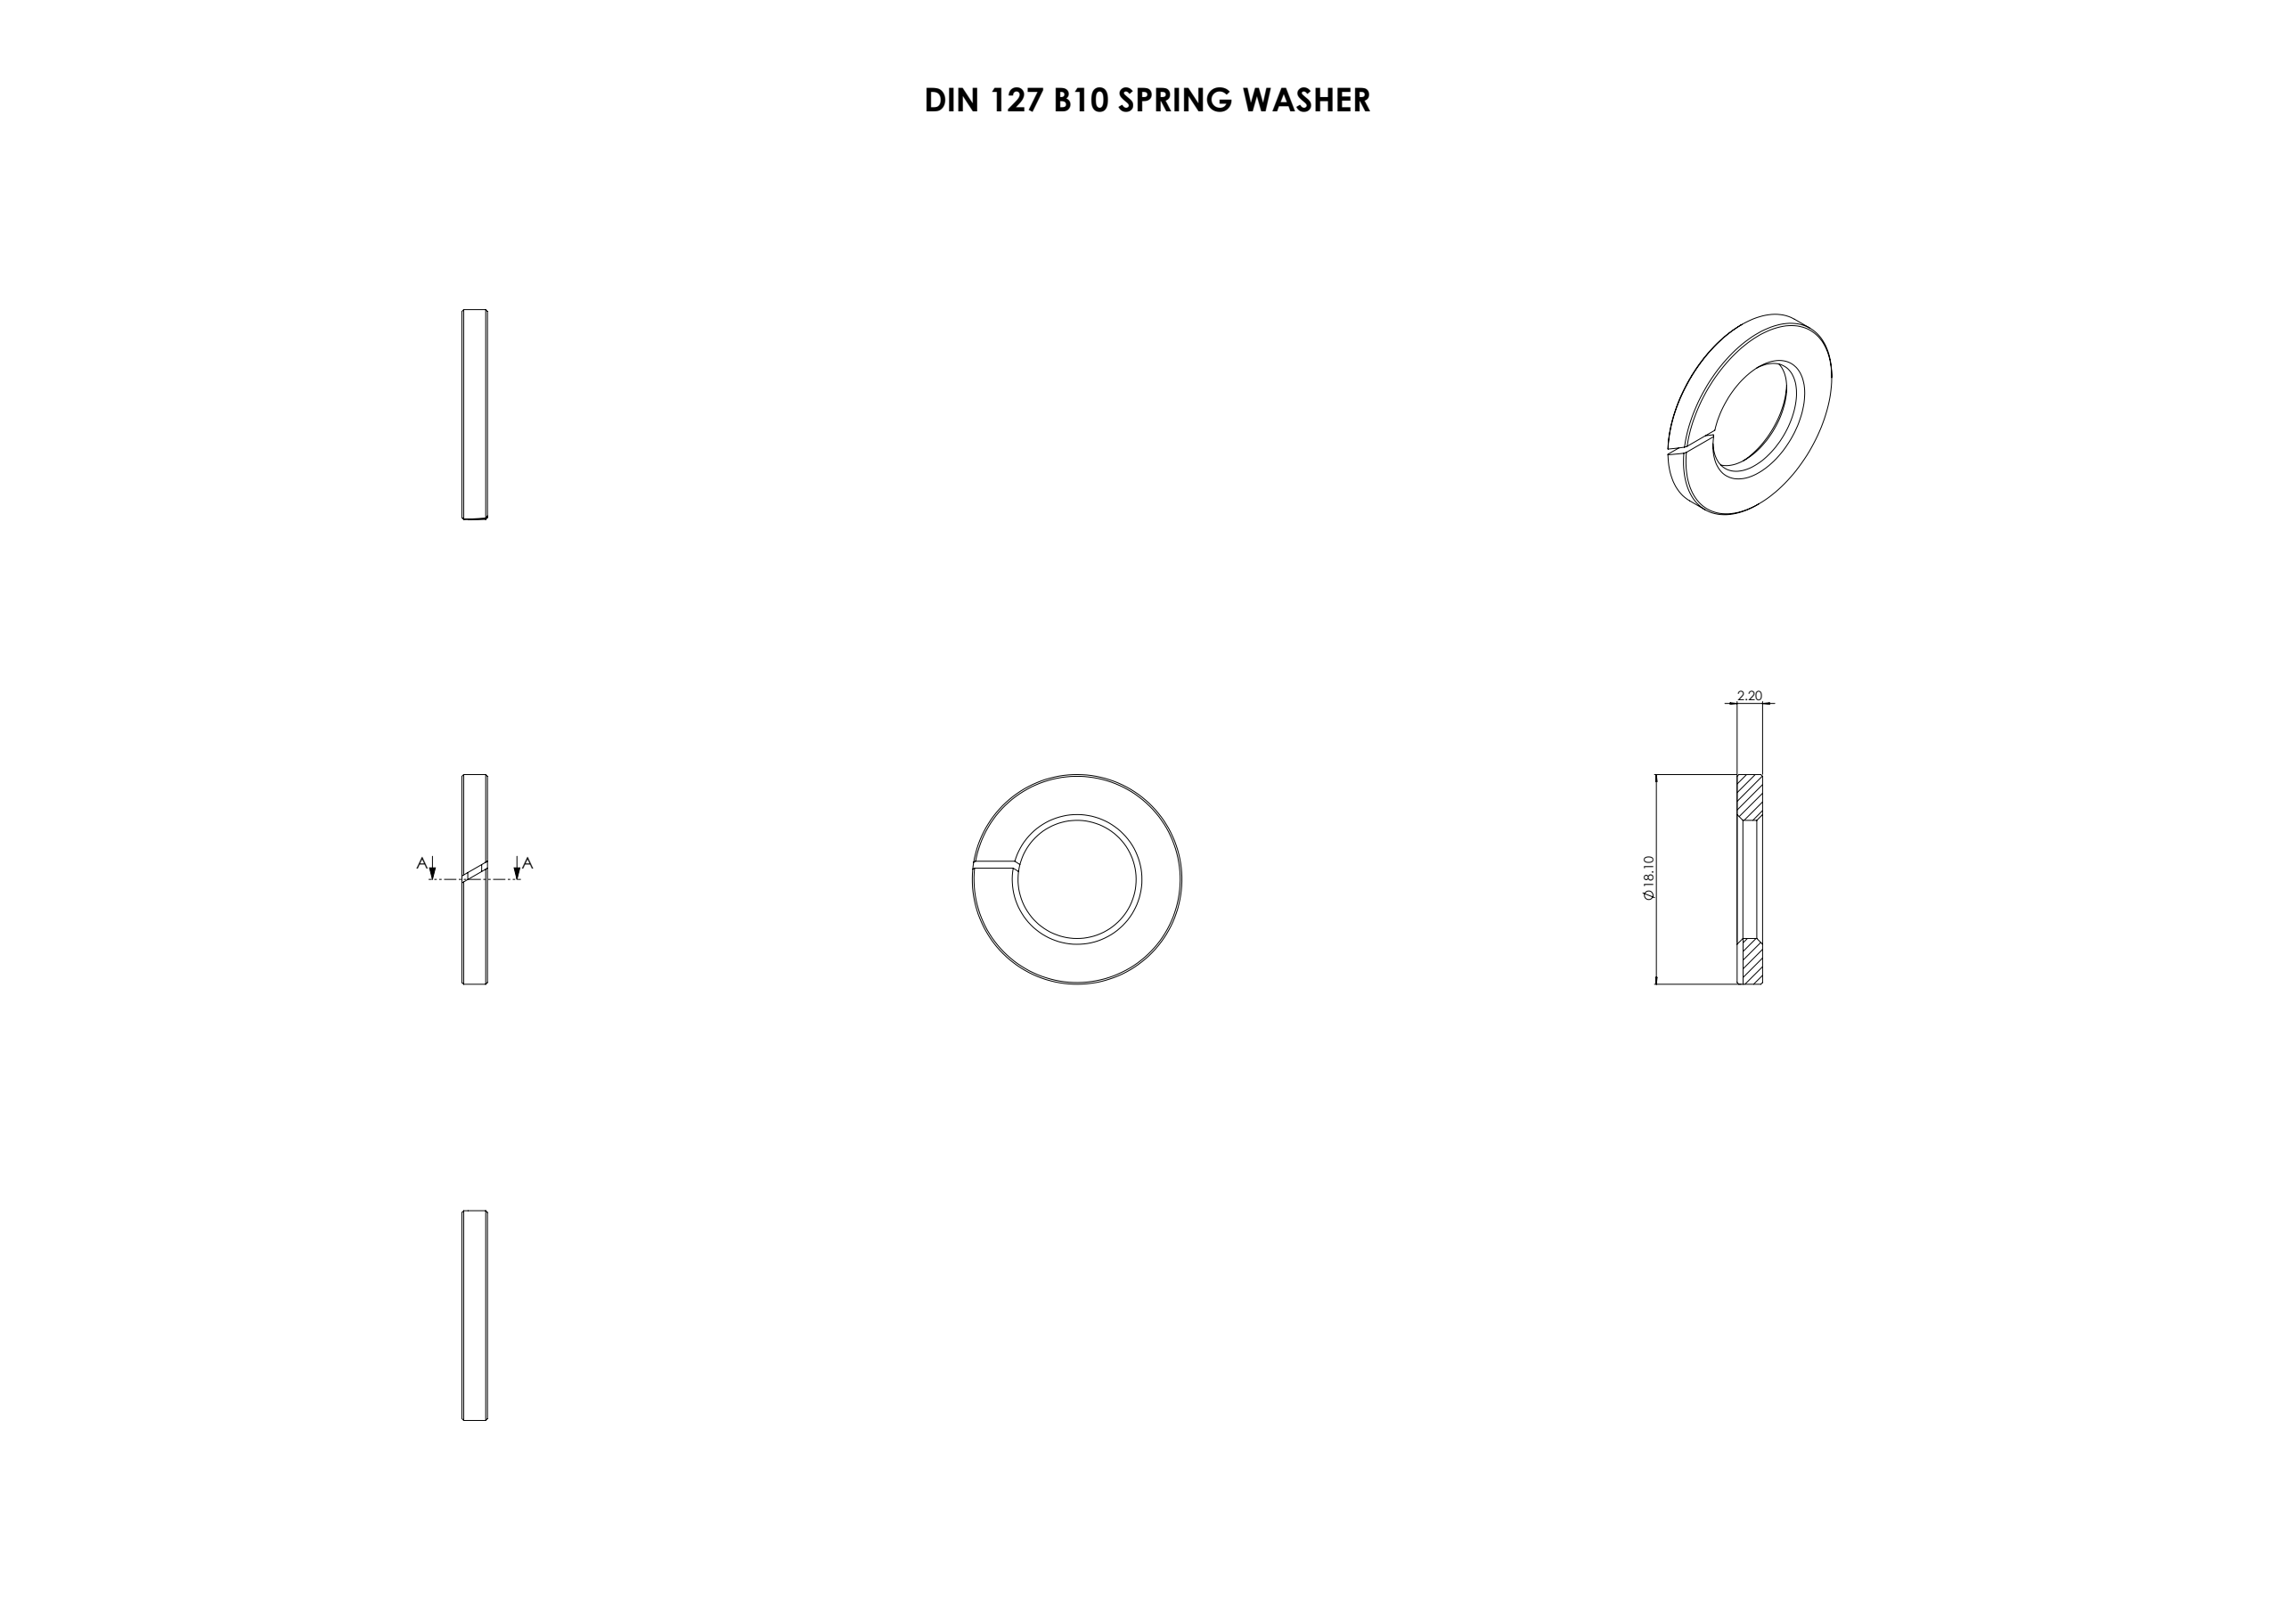
ISO-10303-21;
HEADER;
/* Generated by software containing ST-Developer
 * from STEP Tools, Inc. (www.steptools.com) 
 */

FILE_DESCRIPTION(
/* description */ (''),
/* implementation_level */ '2;1');

FILE_NAME(
/* name */ '08_DIN_127_B10_Spring_Washer.step',
/* time_stamp */ '2026-10-11T08:27:52-07:00',
/* author */ (''),
/* organization */ (''),
/* preprocessor_version */ 'ST-DEVELOPER v20.2',
/* originating_system */ 'Autodesk Translation Framework v15.15.0.0',
/* authorisation */ '');

FILE_SCHEMA (('AUTOMOTIVE_DESIGN { 1 0 10303 214 3 1 1 }'));
ENDSEC;

DATA;
#10=MECHANICAL_DESIGN_GEOMETRIC_PRESENTATION_REPRESENTATION('',(#926),#94301);
#898=SHAPE_REPRESENTATION_RELATIONSHIP('SRR','None',#94378,#912);
#912=ADVANCED_BREP_SHAPE_REPRESENTATION('',(#940),#94294);
#926=STYLED_ITEM('',(#94588),#940);
#940=MANIFOLD_SOLID_BREP('Body1',#51025);
#1194=CYLINDRICAL_SURFACE('',#54830,5.1);
#1195=CYLINDRICAL_SURFACE('',#54834,9.05);
#1196=CYLINDRICAL_SURFACE('',#54845,9.05);
#1197=CYLINDRICAL_SURFACE('',#54853,5.1);
#2152=ELLIPSE('',#54832,10.2,5.1);
#2153=ELLIPSE('',#54836,18.1,9.05);
#2154=ELLIPSE('',#54839,18.1,9.05);
#2155=ELLIPSE('',#54841,10.2,5.1);
#6291=LINE('',#87401,#10819);
#6292=LINE('',#87410,#10820);
#6293=LINE('',#87422,#10821);
#6294=LINE('',#87434,#10822);
#6295=LINE('',#87451,#10823);
#6296=LINE('',#87459,#10824);
#10819=VECTOR('',#66787,5.1);
#10820=VECTOR('',#66796,9.05);
#10821=VECTOR('',#66805,10.);
#10822=VECTOR('',#66808,10.);
#10823=VECTOR('',#66813,10.);
#10824=VECTOR('',#66814,10.);
#13061=PLANE('',#54838);
#13062=PLANE('',#54840);
#13063=PLANE('',#54849);
#13064=PLANE('',#54857);
#15619=FACE_OUTER_BOUND('',#18377,.T.);
#15620=FACE_OUTER_BOUND('',#18378,.T.);
#15621=FACE_OUTER_BOUND('',#18379,.T.);
#15622=FACE_OUTER_BOUND('',#18380,.T.);
#15623=FACE_OUTER_BOUND('',#18381,.T.);
#15624=FACE_OUTER_BOUND('',#18382,.T.);
#15625=FACE_OUTER_BOUND('',#18383,.T.);
#15626=FACE_OUTER_BOUND('',#18384,.T.);
#15627=FACE_OUTER_BOUND('',#18385,.T.);
#15628=FACE_OUTER_BOUND('',#18386,.T.);
#15629=FACE_OUTER_BOUND('',#18387,.T.);
#15630=FACE_OUTER_BOUND('',#18388,.T.);
#18377=EDGE_LOOP('',(#46535,#46536,#46537,#46538));
#18378=EDGE_LOOP('',(#46539,#46540,#46541,#46542));
#18379=EDGE_LOOP('',(#46543,#46544,#46545,#46546,#46547,#46548,#46549,#46550));
#18380=EDGE_LOOP('',(#46551,#46552,#46553,#46554,#46555,#46556,#46557,#46558));
#18381=EDGE_LOOP('',(#46559,#46560,#46561,#46562,#46563));
#18382=EDGE_LOOP('',(#46564,#46565,#46566,#46567));
#18383=EDGE_LOOP('',(#46568,#46569,#46570,#46571,#46572));
#18384=EDGE_LOOP('',(#46573,#46574,#46575,#46576));
#18385=EDGE_LOOP('',(#46577,#46578,#46579,#46580,#46581));
#18386=EDGE_LOOP('',(#46582,#46583,#46584,#46585));
#18387=EDGE_LOOP('',(#46586,#46587,#46588,#46589,#46590));
#18388=EDGE_LOOP('',(#46591,#46592,#46593,#46594));
#19540=(
BOUNDED_CURVE()
B_SPLINE_CURVE(2,(#87418,#87419,#87420),.UNSPECIFIED.,.F.,.F.)
B_SPLINE_CURVE_WITH_KNOTS((3,3),(0.,0.0725293307675455),.UNSPECIFIED.)
CURVE()
GEOMETRIC_REPRESENTATION_ITEM()
RATIONAL_B_SPLINE_CURVE((1.,1.00078463175291,1.))
REPRESENTATION_ITEM('')
);
#19541=(
BOUNDED_CURVE()
B_SPLINE_CURVE(2,(#87424,#87425,#87426),.UNSPECIFIED.,.F.,.F.)
B_SPLINE_CURVE_WITH_KNOTS((3,3),(0.,0.0240722006597559),.UNSPECIFIED.)
CURVE()
GEOMETRIC_REPRESENTATION_ITEM()
RATIONAL_B_SPLINE_CURVE((1.,1.00002397294334,1.))
REPRESENTATION_ITEM('')
);
#19542=(
BOUNDED_CURVE()
B_SPLINE_CURVE(2,(#87430,#87431,#87432),.UNSPECIFIED.,.F.,.F.)
B_SPLINE_CURVE_WITH_KNOTS((3,3),(0.,0.022704443195243),.UNSPECIFIED.)
CURVE()
GEOMETRIC_REPRESENTATION_ITEM()
RATIONAL_B_SPLINE_CURVE((1.,1.00002331266599,1.))
REPRESENTATION_ITEM('')
);
#19543=(
BOUNDED_CURVE()
B_SPLINE_CURVE(2,(#87435,#87436,#87437),.UNSPECIFIED.,.F.,.F.)
B_SPLINE_CURVE_WITH_KNOTS((3,3),(0.,0.0781071789666387),.UNSPECIFIED.)
CURVE()
GEOMETRIC_REPRESENTATION_ITEM()
RATIONAL_B_SPLINE_CURVE((1.,1.00073443968728,1.))
REPRESENTATION_ITEM('')
);
#19544=(
BOUNDED_CURVE()
B_SPLINE_CURVE(2,(#87441,#87442,#87443),.UNSPECIFIED.,.F.,.F.)
B_SPLINE_CURVE_WITH_KNOTS((3,3),(0.,0.0738858532870895),.UNSPECIFIED.)
CURVE()
GEOMETRIC_REPRESENTATION_ITEM()
RATIONAL_B_SPLINE_CURVE((1.,1.00074677418322,1.))
REPRESENTATION_ITEM('')
);
#19545=(
BOUNDED_CURVE()
B_SPLINE_CURVE(2,(#87447,#87448,#87449),.UNSPECIFIED.,.F.,.F.)
B_SPLINE_CURVE_WITH_KNOTS((3,3),(0.,0.0758535488683919),.UNSPECIFIED.)
CURVE()
GEOMETRIC_REPRESENTATION_ITEM()
RATIONAL_B_SPLINE_CURVE((1.,1.00072976064601,1.))
REPRESENTATION_ITEM('')
);
#19546=(
BOUNDED_CURVE()
B_SPLINE_CURVE(2,(#87452,#87453,#87454),.UNSPECIFIED.,.F.,.F.)
B_SPLINE_CURVE_WITH_KNOTS((3,3),(0.,0.0230800535081001),.UNSPECIFIED.)
CURVE()
GEOMETRIC_REPRESENTATION_ITEM()
RATIONAL_B_SPLINE_CURVE((1.,1.0000232977523,1.))
REPRESENTATION_ITEM('')
);
#19547=(
BOUNDED_CURVE()
B_SPLINE_CURVE(2,(#87456,#87457,#87458),.UNSPECIFIED.,.F.,.F.)
B_SPLINE_CURVE_WITH_KNOTS((3,3),(0.,0.0235661439474371),.UNSPECIFIED.)
CURVE()
GEOMETRIC_REPRESENTATION_ITEM()
RATIONAL_B_SPLINE_CURVE((1.,1.00002352982172,1.))
REPRESENTATION_ITEM('')
);
#20142=CIRCLE('',#54831,5.1);
#20143=CIRCLE('',#54833,5.1);
#20144=CIRCLE('',#54835,9.05);
#20145=CIRCLE('',#54837,9.05);
#20146=CIRCLE('',#54843,9.05);
#20147=CIRCLE('',#54844,8.9);
#20148=CIRCLE('',#54846,9.05);
#20149=CIRCLE('',#54848,8.9);
#20150=CIRCLE('',#54850,5.6);
#20151=CIRCLE('',#54852,5.1);
#20152=CIRCLE('',#54854,5.1);
#20153=CIRCLE('',#54856,5.6);
#24824=VERTEX_POINT('',#87399);
#24825=VERTEX_POINT('',#87400);
#24826=VERTEX_POINT('',#87402);
#24827=VERTEX_POINT('',#87404);
#24828=VERTEX_POINT('',#87408);
#24829=VERTEX_POINT('',#87409);
#24830=VERTEX_POINT('',#87411);
#24831=VERTEX_POINT('',#87413);
#24832=VERTEX_POINT('',#87417);
#24833=VERTEX_POINT('',#87421);
#24834=VERTEX_POINT('',#87423);
#24835=VERTEX_POINT('',#87427);
#24836=VERTEX_POINT('',#87429);
#24837=VERTEX_POINT('',#87433);
#24838=VERTEX_POINT('',#87439);
#24839=VERTEX_POINT('',#87440);
#24840=VERTEX_POINT('',#87444);
#24841=VERTEX_POINT('',#87446);
#24842=VERTEX_POINT('',#87450);
#24843=VERTEX_POINT('',#87455);
#32129=EDGE_CURVE('',#24824,#24825,#6291,.T.);
#32130=EDGE_CURVE('',#24826,#24824,#20142,.T.);
#32131=EDGE_CURVE('',#24826,#24827,#2152,.T.);
#32132=EDGE_CURVE('',#24825,#24827,#20143,.T.);
#32133=EDGE_CURVE('',#24828,#24829,#6292,.T.);
#32134=EDGE_CURVE('',#24830,#24828,#20144,.T.);
#32135=EDGE_CURVE('',#24830,#24831,#2153,.T.);
#32136=EDGE_CURVE('',#24829,#24831,#20145,.T.);
#32137=EDGE_CURVE('',#24832,#24826,#19540,.T.);
#32138=EDGE_CURVE('',#24833,#24832,#6293,.T.);
#32139=EDGE_CURVE('',#24834,#24833,#19541,.T.);
#32140=EDGE_CURVE('',#24835,#24834,#2154,.T.);
#32141=EDGE_CURVE('',#24836,#24835,#19542,.T.);
#32142=EDGE_CURVE('',#24837,#24836,#6294,.T.);
#32143=EDGE_CURVE('',#24827,#24837,#19543,.T.);
#32144=EDGE_CURVE('',#24838,#24839,#19544,.T.);
#32145=EDGE_CURVE('',#24840,#24838,#2155,.T.);
#32146=EDGE_CURVE('',#24841,#24840,#19545,.T.);
#32147=EDGE_CURVE('',#24842,#24841,#6295,.T.);
#32148=EDGE_CURVE('',#24831,#24842,#19546,.T.);
#32149=EDGE_CURVE('',#24843,#24830,#19547,.T.);
#32150=EDGE_CURVE('',#24839,#24843,#6296,.T.);
#32151=EDGE_CURVE('',#24835,#24829,#20146,.T.);
#32152=EDGE_CURVE('',#24842,#24836,#20147,.T.);
#32153=EDGE_CURVE('',#24828,#24834,#20148,.T.);
#32154=EDGE_CURVE('',#24833,#24843,#20149,.T.);
#32155=EDGE_CURVE('',#24839,#24832,#20150,.T.);
#32156=EDGE_CURVE('',#24824,#24838,#20151,.T.);
#32157=EDGE_CURVE('',#24840,#24825,#20152,.T.);
#32158=EDGE_CURVE('',#24837,#24841,#20153,.T.);
#46535=ORIENTED_EDGE('',*,*,#32129,.F.);
#46536=ORIENTED_EDGE('',*,*,#32130,.F.);
#46537=ORIENTED_EDGE('',*,*,#32131,.T.);
#46538=ORIENTED_EDGE('',*,*,#32132,.F.);
#46539=ORIENTED_EDGE('',*,*,#32133,.F.);
#46540=ORIENTED_EDGE('',*,*,#32134,.F.);
#46541=ORIENTED_EDGE('',*,*,#32135,.T.);
#46542=ORIENTED_EDGE('',*,*,#32136,.F.);
#46543=ORIENTED_EDGE('',*,*,#32137,.F.);
#46544=ORIENTED_EDGE('',*,*,#32138,.F.);
#46545=ORIENTED_EDGE('',*,*,#32139,.F.);
#46546=ORIENTED_EDGE('',*,*,#32140,.F.);
#46547=ORIENTED_EDGE('',*,*,#32141,.F.);
#46548=ORIENTED_EDGE('',*,*,#32142,.F.);
#46549=ORIENTED_EDGE('',*,*,#32143,.F.);
#46550=ORIENTED_EDGE('',*,*,#32131,.F.);
#46551=ORIENTED_EDGE('',*,*,#32144,.F.);
#46552=ORIENTED_EDGE('',*,*,#32145,.F.);
#46553=ORIENTED_EDGE('',*,*,#32146,.F.);
#46554=ORIENTED_EDGE('',*,*,#32147,.F.);
#46555=ORIENTED_EDGE('',*,*,#32148,.F.);
#46556=ORIENTED_EDGE('',*,*,#32135,.F.);
#46557=ORIENTED_EDGE('',*,*,#32149,.F.);
#46558=ORIENTED_EDGE('',*,*,#32150,.F.);
#46559=ORIENTED_EDGE('',*,*,#32141,.T.);
#46560=ORIENTED_EDGE('',*,*,#32151,.T.);
#46561=ORIENTED_EDGE('',*,*,#32136,.T.);
#46562=ORIENTED_EDGE('',*,*,#32148,.T.);
#46563=ORIENTED_EDGE('',*,*,#32152,.T.);
#46564=ORIENTED_EDGE('',*,*,#32133,.T.);
#46565=ORIENTED_EDGE('',*,*,#32151,.F.);
#46566=ORIENTED_EDGE('',*,*,#32140,.T.);
#46567=ORIENTED_EDGE('',*,*,#32153,.F.);
#46568=ORIENTED_EDGE('',*,*,#32139,.T.);
#46569=ORIENTED_EDGE('',*,*,#32154,.T.);
#46570=ORIENTED_EDGE('',*,*,#32149,.T.);
#46571=ORIENTED_EDGE('',*,*,#32134,.T.);
#46572=ORIENTED_EDGE('',*,*,#32153,.T.);
#46573=ORIENTED_EDGE('',*,*,#32138,.T.);
#46574=ORIENTED_EDGE('',*,*,#32155,.F.);
#46575=ORIENTED_EDGE('',*,*,#32150,.T.);
#46576=ORIENTED_EDGE('',*,*,#32154,.F.);
#46577=ORIENTED_EDGE('',*,*,#32137,.T.);
#46578=ORIENTED_EDGE('',*,*,#32130,.T.);
#46579=ORIENTED_EDGE('',*,*,#32156,.T.);
#46580=ORIENTED_EDGE('',*,*,#32144,.T.);
#46581=ORIENTED_EDGE('',*,*,#32155,.T.);
#46582=ORIENTED_EDGE('',*,*,#32129,.T.);
#46583=ORIENTED_EDGE('',*,*,#32157,.F.);
#46584=ORIENTED_EDGE('',*,*,#32145,.T.);
#46585=ORIENTED_EDGE('',*,*,#32156,.F.);
#46586=ORIENTED_EDGE('',*,*,#32143,.T.);
#46587=ORIENTED_EDGE('',*,*,#32158,.T.);
#46588=ORIENTED_EDGE('',*,*,#32146,.T.);
#46589=ORIENTED_EDGE('',*,*,#32157,.T.);
#46590=ORIENTED_EDGE('',*,*,#32132,.T.);
#46591=ORIENTED_EDGE('',*,*,#32142,.T.);
#46592=ORIENTED_EDGE('',*,*,#32152,.F.);
#46593=ORIENTED_EDGE('',*,*,#32147,.T.);
#46594=ORIENTED_EDGE('',*,*,#32158,.F.);
#48313=CONICAL_SURFACE('',#54842,8.975,0.785398163397449);
#48314=CONICAL_SURFACE('',#54847,8.975,0.785398163397448);
#48315=CONICAL_SURFACE('',#54851,5.35,0.785398163397449);
#48316=CONICAL_SURFACE('',#54855,5.35,0.785398163397449);
#50706=ADVANCED_FACE('',(#15619),#1194,.F.);
#50707=ADVANCED_FACE('',(#15620),#1195,.T.);
#50708=ADVANCED_FACE('',(#15621),#13061,.F.);
#50709=ADVANCED_FACE('',(#15622),#13062,.F.);
#50710=ADVANCED_FACE('',(#15623),#48313,.T.);
#50711=ADVANCED_FACE('',(#15624),#1196,.T.);
#50712=ADVANCED_FACE('',(#15625),#48314,.T.);
#50713=ADVANCED_FACE('',(#15626),#13063,.T.);
#50714=ADVANCED_FACE('',(#15627),#48315,.F.);
#50715=ADVANCED_FACE('',(#15628),#1197,.F.);
#50716=ADVANCED_FACE('',(#15629),#48316,.F.);
#50717=ADVANCED_FACE('',(#15630),#13064,.T.);
#51025=CLOSED_SHELL('',(#50706,#50707,#50708,#50709,#50710,#50711,#50712,
#50713,#50714,#50715,#50716,#50717));
#54829=AXIS2_PLACEMENT_3D('',#87397,#66783,#66784);
#54830=AXIS2_PLACEMENT_3D('',#87398,#66785,#66786);
#54831=AXIS2_PLACEMENT_3D('',#87403,#66788,#66789);
#54832=AXIS2_PLACEMENT_3D('',#87405,#66790,#66791);
#54833=AXIS2_PLACEMENT_3D('',#87406,#66792,#66793);
#54834=AXIS2_PLACEMENT_3D('',#87407,#66794,#66795);
#54835=AXIS2_PLACEMENT_3D('',#87412,#66797,#66798);
#54836=AXIS2_PLACEMENT_3D('',#87414,#66799,#66800);
#54837=AXIS2_PLACEMENT_3D('',#87415,#66801,#66802);
#54838=AXIS2_PLACEMENT_3D('',#87416,#66803,#66804);
#54839=AXIS2_PLACEMENT_3D('',#87428,#66806,#66807);
#54840=AXIS2_PLACEMENT_3D('',#87438,#66809,#66810);
#54841=AXIS2_PLACEMENT_3D('',#87445,#66811,#66812);
#54842=AXIS2_PLACEMENT_3D('',#87460,#66815,#66816);
#54843=AXIS2_PLACEMENT_3D('',#87461,#66817,#66818);
#54844=AXIS2_PLACEMENT_3D('',#87462,#66819,#66820);
#54845=AXIS2_PLACEMENT_3D('',#87463,#66821,#66822);
#54846=AXIS2_PLACEMENT_3D('',#87464,#66823,#66824);
#54847=AXIS2_PLACEMENT_3D('',#87465,#66825,#66826);
#54848=AXIS2_PLACEMENT_3D('',#87466,#66827,#66828);
#54849=AXIS2_PLACEMENT_3D('',#87467,#66829,#66830);
#54850=AXIS2_PLACEMENT_3D('',#87468,#66831,#66832);
#54851=AXIS2_PLACEMENT_3D('',#87469,#66833,#66834);
#54852=AXIS2_PLACEMENT_3D('',#87470,#66835,#66836);
#54853=AXIS2_PLACEMENT_3D('',#87471,#66837,#66838);
#54854=AXIS2_PLACEMENT_3D('',#87472,#66839,#66840);
#54855=AXIS2_PLACEMENT_3D('',#87473,#66841,#66842);
#54856=AXIS2_PLACEMENT_3D('',#87474,#66843,#66844);
#54857=AXIS2_PLACEMENT_3D('',#87475,#66845,#66846);
#66783=DIRECTION('axis',(0.,0.,1.));
#66784=DIRECTION('refdir',(1.,0.,0.));
#66785=DIRECTION('center_axis',(1.,0.,0.));
#66786=DIRECTION('ref_axis',(0.,1.,0.));
#66787=DIRECTION('',(-1.,0.,0.));
#66788=DIRECTION('center_axis',(-1.,0.,0.));
#66789=DIRECTION('ref_axis',(0.,-1.,0.));
#66790=DIRECTION('center_axis',(0.5,-0.866025403784439,0.));
#66791=DIRECTION('ref_axis',(0.866025403784439,0.5,0.));
#66792=DIRECTION('center_axis',(1.,0.,0.));
#66793=DIRECTION('ref_axis',(0.,-1.,0.));
#66794=DIRECTION('center_axis',(1.,0.,0.));
#66795=DIRECTION('ref_axis',(0.,1.,0.));
#66796=DIRECTION('',(-1.,0.,0.));
#66797=DIRECTION('center_axis',(1.,0.,0.));
#66798=DIRECTION('ref_axis',(0.,-1.,0.));
#66799=DIRECTION('center_axis',(0.5,-0.866025403784439,0.));
#66800=DIRECTION('ref_axis',(0.866025403784439,0.5,0.));
#66801=DIRECTION('center_axis',(-1.,0.,0.));
#66802=DIRECTION('ref_axis',(0.,-1.,0.));
#66803=DIRECTION('center_axis',(-0.5,0.866025403784439,0.));
#66804=DIRECTION('ref_axis',(-0.866025403784439,-0.5,0.));
#66805=DIRECTION('',(0.,0.,-1.));
#66806=DIRECTION('center_axis',(-0.5,0.866025403784439,0.));
#66807=DIRECTION('ref_axis',(0.866025403784439,0.5,0.));
#66808=DIRECTION('',(0.,0.,1.));
#66809=DIRECTION('center_axis',(0.5,-0.866025403784439,0.));
#66810=DIRECTION('ref_axis',(0.866025403784439,0.5,0.));
#66811=DIRECTION('center_axis',(-0.5,0.866025403784439,0.));
#66812=DIRECTION('ref_axis',(0.866025403784439,0.5,0.));
#66813=DIRECTION('',(0.,0.,-1.));
#66814=DIRECTION('',(0.,0.,1.));
#66815=DIRECTION('center_axis',(1.,0.,0.));
#66816=DIRECTION('ref_axis',(0.,-0.00506609645795909,-0.999987167251));
#66817=DIRECTION('center_axis',(-1.,0.,0.));
#66818=DIRECTION('ref_axis',(0.,-1.,0.));
#66819=DIRECTION('center_axis',(1.,0.,0.));
#66820=DIRECTION('ref_axis',(0.,-1.,0.));
#66821=DIRECTION('center_axis',(1.,0.,0.));
#66822=DIRECTION('ref_axis',(0.,1.,0.));
#66823=DIRECTION('center_axis',(1.,0.,0.));
#66824=DIRECTION('ref_axis',(0.,-1.,0.));
#66825=DIRECTION('center_axis',(-1.,0.,0.));
#66826=DIRECTION('ref_axis',(0.,-0.13652151564835,-0.990637105990421));
#66827=DIRECTION('center_axis',(-1.,0.,0.));
#66828=DIRECTION('ref_axis',(0.,-1.,0.));
#66829=DIRECTION('center_axis',(1.,0.,0.));
#66830=DIRECTION('ref_axis',(0.,0.,-1.));
#66831=DIRECTION('center_axis',(1.,0.,0.));
#66832=DIRECTION('ref_axis',(0.,-1.,0.));
#66833=DIRECTION('center_axis',(1.,0.,0.));
#66834=DIRECTION('ref_axis',(0.,-0.212428563289972,-0.977176598931103));
#66835=DIRECTION('center_axis',(-1.,0.,0.));
#66836=DIRECTION('ref_axis',(0.,-1.,0.));
#66837=DIRECTION('center_axis',(1.,0.,0.));
#66838=DIRECTION('ref_axis',(0.,1.,0.));
#66839=DIRECTION('center_axis',(1.,0.,0.));
#66840=DIRECTION('ref_axis',(0.,-1.,0.));
#66841=DIRECTION('center_axis',(-1.,0.,0.));
#66842=DIRECTION('ref_axis',(0.,-0.0256854359394706,-0.999670074764969));
#66843=DIRECTION('center_axis',(-1.,0.,0.));
#66844=DIRECTION('ref_axis',(0.,-1.,0.));
#66845=DIRECTION('center_axis',(-1.,0.,0.));
#66846=DIRECTION('ref_axis',(0.,0.,1.));
#87397=CARTESIAN_POINT('',(0.,0.,0.));
#87398=CARTESIAN_POINT('Origin',(1.1,0.,0.));
#87399=CARTESIAN_POINT('',(1.7,-5.1,-6.2456986756515E-16));
#87400=CARTESIAN_POINT('',(0.499999999999998,-5.1,-6.2456986756515E-16));
#87401=CARTESIAN_POINT('',(1.1,-5.1,-6.2456986756515E-16));
#87402=CARTESIAN_POINT('',(1.7,1.28149545762236,4.93637208809195));
#87403=CARTESIAN_POINT('Origin',(1.7,0.,0.));
#87404=CARTESIAN_POINT('',(0.5,0.588675134594813,5.06591172306721));
#87405=CARTESIAN_POINT('Origin',(-0.519615242270663,0.,0.));
#87406=CARTESIAN_POINT('Origin',(0.5,0.,0.));
#87407=CARTESIAN_POINT('Origin',(1.1,0.,0.));
#87408=CARTESIAN_POINT('',(2.05,-9.05,-1.10830535322835E-15));
#87409=CARTESIAN_POINT('',(0.149999999999998,-9.05,-1.10830535322835E-15));
#87410=CARTESIAN_POINT('',(1.1,-9.05,-1.10830535322835E-15));
#87411=CARTESIAN_POINT('',(2.05,0.883568051838733,9.00676454104191));
#87412=CARTESIAN_POINT('Origin',(2.05,0.,0.));
#87413=CARTESIAN_POINT('',(0.15,-0.213397459621556,9.0474837122941));
#87414=CARTESIAN_POINT('Origin',(0.519615242270663,0.,0.));
#87415=CARTESIAN_POINT('Origin',(0.15,0.,0.));
#87416=CARTESIAN_POINT('Origin',(2.4,1.6856406460551,0.));
#87417=CARTESIAN_POINT('',(2.2,1.57017059221718,5.37536643507551));
#87418=CARTESIAN_POINT('Ctrl Pts',(2.2,1.57017059221718,5.37536643507551));
#87419=CARTESIAN_POINT('Ctrl Pts',(1.93935692691251,1.4196882438077,5.14778785676925));
#87420=CARTESIAN_POINT('Ctrl Pts',(1.7,1.28149545762236,4.93637208809195));
#87421=CARTESIAN_POINT('',(2.2,1.57017059221718,8.76039749733631));
#87422=CARTESIAN_POINT('',(2.2,1.57017059221718,0.));
#87423=CARTESIAN_POINT('',(2.05,1.48356805183873,8.92757110504103));
#87424=CARTESIAN_POINT('Ctrl Pts',(2.05,1.48356805183873,8.92757110504103));
#87425=CARTESIAN_POINT('Ctrl Pts',(2.12570884457451,1.52727857363386,8.84356028415378));
#87426=CARTESIAN_POINT('Ctrl Pts',(2.2,1.57017059221718,8.76039749733631));
#87427=CARTESIAN_POINT('',(0.15,0.386602540378444,9.04173868654547));
#87428=CARTESIAN_POINT('Origin',(-0.519615242270663,0.,0.));
#87429=CARTESIAN_POINT('',(0.,0.3,8.89494238317483));
#87430=CARTESIAN_POINT('Ctrl Pts',(0.,0.3,8.89494238317483));
#87431=CARTESIAN_POINT('Ctrl Pts',(0.0743861895232588,0.342946886545244,
8.96792239730301));
#87432=CARTESIAN_POINT('Ctrl Pts',(0.15,0.386602540378444,9.04173868654547));
#87433=CARTESIAN_POINT('',(0.,0.3,5.59195851200633));
#87434=CARTESIAN_POINT('',(5.55111512312578E-16,0.299999999999999,0.));
#87435=CARTESIAN_POINT('Ctrl Pts',(0.5,0.588675134594813,5.06591172306721));
#87436=CARTESIAN_POINT('Ctrl Pts',(0.262339397490468,0.451461721760166,
5.32111616952063));
#87437=CARTESIAN_POINT('Ctrl Pts',(0.,0.3,5.59195851200633));
#87438=CARTESIAN_POINT('Origin',(-0.2,-0.415470053837925,0.));
#87439=CARTESIAN_POINT('',(1.7,0.681495457622364,5.05426195811417));
#87440=CARTESIAN_POINT('',(2.2,0.970170592217176,5.51532129816541));
#87441=CARTESIAN_POINT('Ctrl Pts',(1.7,0.681495457622364,5.05426195811417));
#87442=CARTESIAN_POINT('Ctrl Pts',(1.93909466606049,0.819536827434189,5.2769073690057));
#87443=CARTESIAN_POINT('Ctrl Pts',(2.2,0.970170592217177,5.51532129816541));
#87444=CARTESIAN_POINT('',(0.5,-0.0113248654051871,5.0999874262025));
#87445=CARTESIAN_POINT('Origin',(0.519615242270663,0.,0.));
#87446=CARTESIAN_POINT('',(0.,-0.3,5.59195851200633));
#87447=CARTESIAN_POINT('Ctrl Pts',(0.,-0.3,5.59195851200633));
#87448=CARTESIAN_POINT('Ctrl Pts',(0.261503310263914,-0.149020993425151,
5.33817894042));
#87449=CARTESIAN_POINT('Ctrl Pts',(0.5,-0.0113248654051871,5.0999874262025));
#87450=CARTESIAN_POINT('',(0.,-0.3,8.89494238317483));
#87451=CARTESIAN_POINT('',(2.77555756156289E-16,-0.3,0.));
#87452=CARTESIAN_POINT('Ctrl Pts',(0.15,-0.213397459621556,9.0474837122941));
#87453=CARTESIAN_POINT('Ctrl Pts',(0.0743623716417539,-0.257066864715054,
8.97079504406147));
#87454=CARTESIAN_POINT('Ctrl Pts',(0.,-0.3,8.89494238317483));
#87455=CARTESIAN_POINT('',(2.2,0.970170592217176,8.84696383071599));
#87456=CARTESIAN_POINT('Ctrl Pts',(2.2,0.970170592217176,8.84696383071599));
#87457=CARTESIAN_POINT('Ctrl Pts',(2.12567129134184,0.927256892264872,8.92644410555483));
#87458=CARTESIAN_POINT('Ctrl Pts',(2.05,0.883568051838733,9.00676454104191));
#87459=CARTESIAN_POINT('',(2.2,0.970170592217176,0.));
#87460=CARTESIAN_POINT('Origin',(0.075,0.,0.));
#87461=CARTESIAN_POINT('Origin',(0.15,0.,0.));
#87462=CARTESIAN_POINT('Origin',(0.,0.,0.));
#87463=CARTESIAN_POINT('Origin',(1.1,0.,0.));
#87464=CARTESIAN_POINT('Origin',(2.05,0.,0.));
#87465=CARTESIAN_POINT('Origin',(2.125,0.,0.));
#87466=CARTESIAN_POINT('Origin',(2.2,0.,0.));
#87467=CARTESIAN_POINT('Origin',(2.2,5.1,0.));
#87468=CARTESIAN_POINT('Origin',(2.2,0.,0.));
#87469=CARTESIAN_POINT('Origin',(1.95,0.,0.));
#87470=CARTESIAN_POINT('Origin',(1.7,0.,0.));
#87471=CARTESIAN_POINT('Origin',(1.1,0.,0.));
#87472=CARTESIAN_POINT('Origin',(0.5,0.,0.));
#87473=CARTESIAN_POINT('Origin',(0.25,0.,0.));
#87474=CARTESIAN_POINT('Origin',(0.,0.,0.));
#87475=CARTESIAN_POINT('Origin',(0.,9.05,0.));
#94278=UNCERTAINTY_MEASURE_WITH_UNIT(LENGTH_MEASURE(0.01),#94302,
'DISTANCE_ACCURACY_VALUE',
'Maximum model space distance between geometric entities at asserted c
onnectivities');
#94285=UNCERTAINTY_MEASURE_WITH_UNIT(LENGTH_MEASURE(0.01),#94302,
'DISTANCE_ACCURACY_VALUE',
'Maximum model space distance between geometric entities at asserted c
onnectivities');
#94294=(
GEOMETRIC_REPRESENTATION_CONTEXT(3)
GLOBAL_UNCERTAINTY_ASSIGNED_CONTEXT((#94278))
GLOBAL_UNIT_ASSIGNED_CONTEXT((#94302,#94304,#94305))
REPRESENTATION_CONTEXT('','3D')
);
#94301=(
GEOMETRIC_REPRESENTATION_CONTEXT(3)
GLOBAL_UNCERTAINTY_ASSIGNED_CONTEXT((#94285))
GLOBAL_UNIT_ASSIGNED_CONTEXT((#94302,#94304,#94305))
REPRESENTATION_CONTEXT('','3D')
);
#94302=(
LENGTH_UNIT()
NAMED_UNIT(*)
SI_UNIT(.MILLI.,.METRE.)
);
#94304=(
NAMED_UNIT(*)
PLANE_ANGLE_UNIT()
SI_UNIT($,.RADIAN.)
);
#94305=(
NAMED_UNIT(*)
SI_UNIT($,.STERADIAN.)
SOLID_ANGLE_UNIT()
);
#94314=SHAPE_DEFINITION_REPRESENTATION(#94329,#94378);
#94329=PRODUCT_DEFINITION_SHAPE('',$,#94394);
#94378=SHAPE_REPRESENTATION('',(#54829),#94294);
#94385=PRODUCT_DEFINITION_CONTEXT('part definition',#94432,'design');
#94394=PRODUCT_DEFINITION('2026-10-11-08-26-40-818',
'08_DIN_127_B10_Spring_Washer',#94409,#94385);
#94409=PRODUCT_DEFINITION_FORMATION('',$,#94442);
#94432=APPLICATION_CONTEXT(
'Core Data for Automotive Mechanical Design Process');
#94433=PRODUCT_CONTEXT('part definition',#94432,'mechanical');
#94442=PRODUCT('2026-10-11-08-26-40-818','08_DIN_127_B10_Spring_Washer',
$,(#94433));
#94582=COLOUR_RGB('Black',0.12,0.14,0.17);
#94583=FILL_AREA_STYLE_COLOUR('',#94582);
#94584=FILL_AREA_STYLE('',(#94583));
#94585=SURFACE_STYLE_FILL_AREA(#94584);
#94586=SURFACE_SIDE_STYLE('',(#94585));
#94587=SURFACE_STYLE_USAGE(.BOTH.,#94586);
#94588=PRESENTATION_STYLE_ASSIGNMENT((#94587));
ENDSEC;
END-ISO-10303-21;
